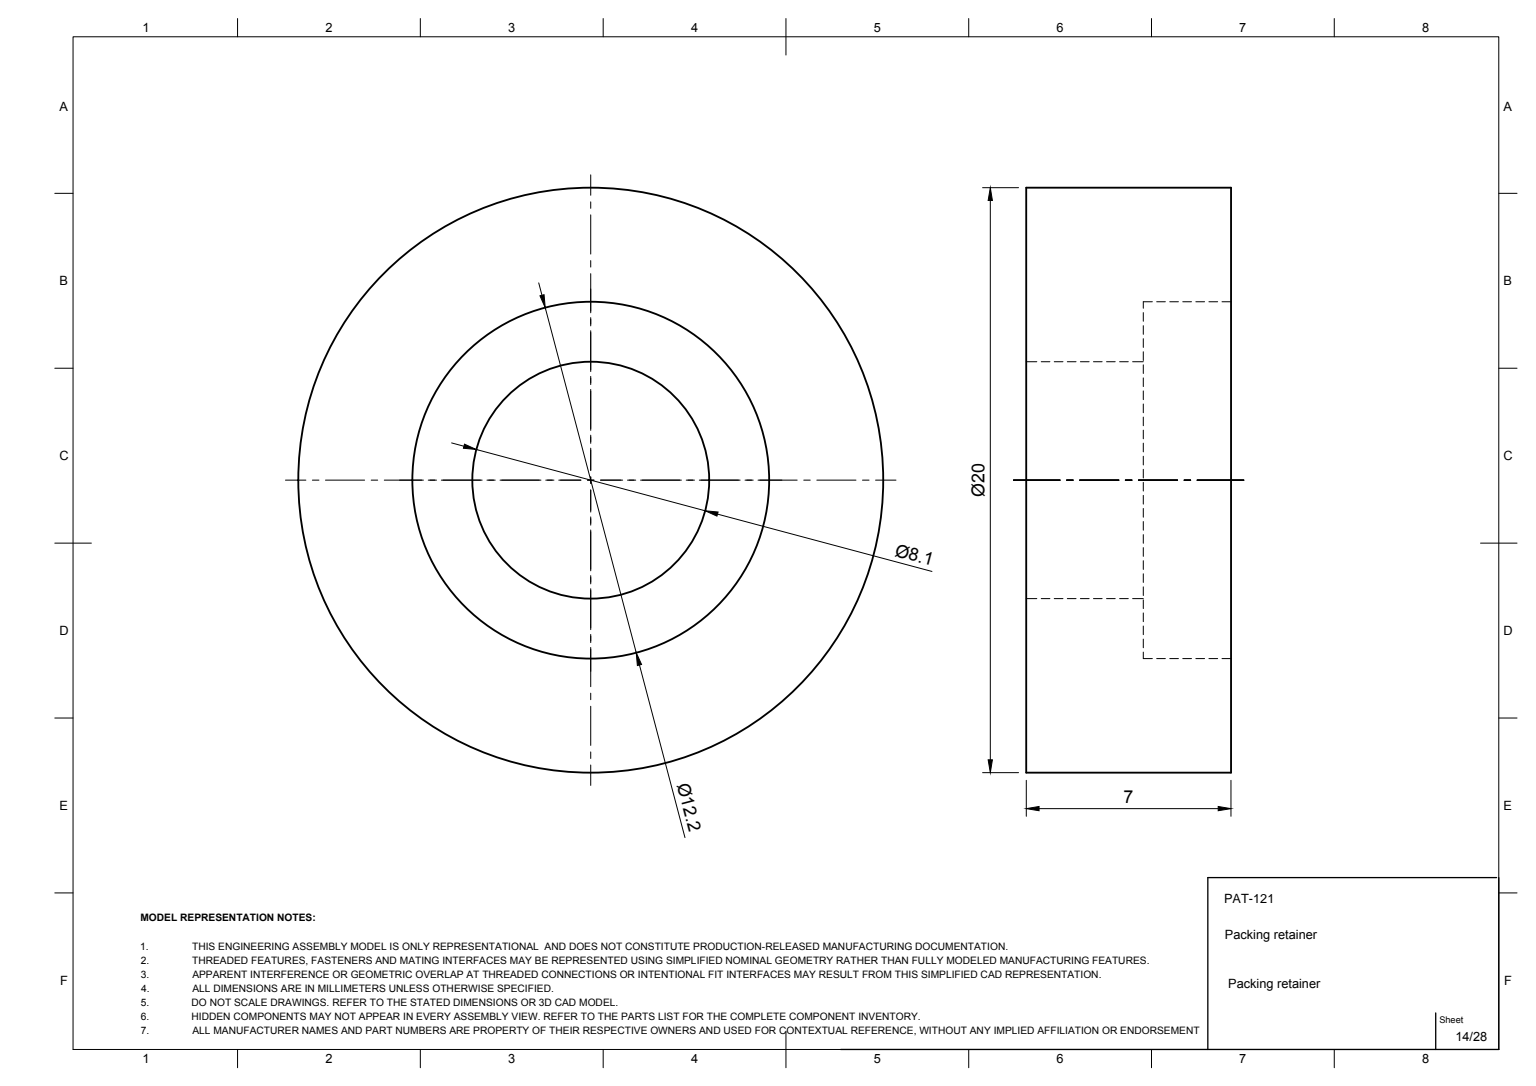
ISO-10303-21;
HEADER;
/* Generated by software containing ST-Developer
 * from STEP Tools, Inc. (www.steptools.com) 
 */

FILE_DESCRIPTION(
/* description */ ('Wall-mounted air drop station'),
/* implementation_level */ '2;1');

FILE_NAME(
/* name */ 'Packing retainer.step',
/* time_stamp */ '2026-10-28T22:16:19-07:00',
/* author */ (''),
/* organization */ (''),
/* preprocessor_version */ 'ST-DEVELOPER v20.2',
/* originating_system */ 'Autodesk Translation Framework v15.17.0.0',
/* authorisation */ '');

FILE_SCHEMA (('AUTOMOTIVE_DESIGN { 1 0 10303 214 3 1 1 }'));
ENDSEC;

DATA;
#10=MECHANICAL_DESIGN_GEOMETRIC_PRESENTATION_REPRESENTATION('',(#354),#10517);
#296=SHAPE_REPRESENTATION_RELATIONSHIP('SRR','None',#10653,#325);
#325=ADVANCED_BREP_SHAPE_REPRESENTATION('',(#383),#10497);
#354=STYLED_ITEM('',(#10860),#383);
#383=MANIFOLD_SOLID_BREP('Body1',#5893);
#474=FACE_BOUND('',#1335,.T.);
#475=FACE_BOUND('',#1339,.T.);
#476=FACE_BOUND('',#1341,.T.);
#616=PLANE('',#6515);
#617=PLANE('',#6522);
#618=PLANE('',#6523);
#903=FACE_OUTER_BOUND('',#1333,.T.);
#904=FACE_OUTER_BOUND('',#1334,.T.);
#905=FACE_OUTER_BOUND('',#1336,.T.);
#906=FACE_OUTER_BOUND('',#1337,.T.);
#907=FACE_OUTER_BOUND('',#1338,.T.);
#908=FACE_OUTER_BOUND('',#1340,.T.);
#1333=EDGE_LOOP('',(#4613,#4614,#4615,#4616));
#1334=EDGE_LOOP('',(#4617));
#1335=EDGE_LOOP('',(#4618));
#1336=EDGE_LOOP('',(#4619,#4620,#4621,#4622));
#1337=EDGE_LOOP('',(#4623,#4624,#4625,#4626));
#1338=EDGE_LOOP('',(#4627));
#1339=EDGE_LOOP('',(#4628));
#1340=EDGE_LOOP('',(#4629));
#1341=EDGE_LOOP('',(#4630));
#1796=LINE('',#9464,#2260);
#1797=LINE('',#9472,#2261);
#1798=LINE('',#9477,#2262);
#2260=VECTOR('',#7686,0.61);
#2261=VECTOR('',#7697,0.405);
#2262=VECTOR('',#7702,1.);
#2636=CIRCLE('',#6513,0.61);
#2637=CIRCLE('',#6514,0.61);
#2638=CIRCLE('',#6516,0.405);
#2639=CIRCLE('',#6518,0.405);
#2640=CIRCLE('',#6520,1.);
#2641=CIRCLE('',#6521,1.);
#2978=VERTEX_POINT('',#9461);
#2979=VERTEX_POINT('',#9463);
#2980=VERTEX_POINT('',#9467);
#2981=VERTEX_POINT('',#9470);
#2982=VERTEX_POINT('',#9474);
#2983=VERTEX_POINT('',#9476);
#3564=EDGE_CURVE('',#2978,#2978,#2636,.T.);
#3565=EDGE_CURVE('',#2978,#2979,#1796,.T.);
#3566=EDGE_CURVE('',#2979,#2979,#2637,.T.);
#3567=EDGE_CURVE('',#2980,#2980,#2638,.T.);
#3568=EDGE_CURVE('',#2981,#2981,#2639,.T.);
#3569=EDGE_CURVE('',#2981,#2980,#1797,.T.);
#3570=EDGE_CURVE('',#2982,#2982,#2640,.T.);
#3571=EDGE_CURVE('',#2982,#2983,#1798,.T.);
#3572=EDGE_CURVE('',#2983,#2983,#2641,.T.);
#4613=ORIENTED_EDGE('',*,*,#3564,.F.);
#4614=ORIENTED_EDGE('',*,*,#3565,.T.);
#4615=ORIENTED_EDGE('',*,*,#3566,.T.);
#4616=ORIENTED_EDGE('',*,*,#3565,.F.);
#4617=ORIENTED_EDGE('',*,*,#3566,.F.);
#4618=ORIENTED_EDGE('',*,*,#3567,.F.);
#4619=ORIENTED_EDGE('',*,*,#3568,.F.);
#4620=ORIENTED_EDGE('',*,*,#3569,.T.);
#4621=ORIENTED_EDGE('',*,*,#3567,.T.);
#4622=ORIENTED_EDGE('',*,*,#3569,.F.);
#4623=ORIENTED_EDGE('',*,*,#3570,.F.);
#4624=ORIENTED_EDGE('',*,*,#3571,.T.);
#4625=ORIENTED_EDGE('',*,*,#3572,.T.);
#4626=ORIENTED_EDGE('',*,*,#3571,.F.);
#4627=ORIENTED_EDGE('',*,*,#3570,.T.);
#4628=ORIENTED_EDGE('',*,*,#3568,.T.);
#4629=ORIENTED_EDGE('',*,*,#3572,.F.);
#4630=ORIENTED_EDGE('',*,*,#3564,.T.);
#5483=CYLINDRICAL_SURFACE('',#6512,0.61);
#5484=CYLINDRICAL_SURFACE('',#6517,0.405);
#5485=CYLINDRICAL_SURFACE('',#6519,1.);
#5676=ADVANCED_FACE('',(#903),#5483,.F.);
#5677=ADVANCED_FACE('',(#904,#474),#616,.F.);
#5678=ADVANCED_FACE('',(#905),#5484,.F.);
#5679=ADVANCED_FACE('',(#906),#5485,.T.);
#5680=ADVANCED_FACE('',(#907,#475),#617,.T.);
#5681=ADVANCED_FACE('',(#908,#476),#618,.F.);
#5893=CLOSED_SHELL('',(#5676,#5677,#5678,#5679,#5680,#5681));
#6511=AXIS2_PLACEMENT_3D('',#9459,#7680,#7681);
#6512=AXIS2_PLACEMENT_3D('',#9460,#7682,#7683);
#6513=AXIS2_PLACEMENT_3D('',#9462,#7684,#7685);
#6514=AXIS2_PLACEMENT_3D('',#9465,#7687,#7688);
#6515=AXIS2_PLACEMENT_3D('',#9466,#7689,#7690);
#6516=AXIS2_PLACEMENT_3D('',#9468,#7691,#7692);
#6517=AXIS2_PLACEMENT_3D('',#9469,#7693,#7694);
#6518=AXIS2_PLACEMENT_3D('',#9471,#7695,#7696);
#6519=AXIS2_PLACEMENT_3D('',#9473,#7698,#7699);
#6520=AXIS2_PLACEMENT_3D('',#9475,#7700,#7701);
#6521=AXIS2_PLACEMENT_3D('',#9478,#7703,#7704);
#6522=AXIS2_PLACEMENT_3D('',#9479,#7705,#7706);
#6523=AXIS2_PLACEMENT_3D('',#9480,#7707,#7708);
#7680=DIRECTION('axis',(0.,0.,1.));
#7681=DIRECTION('refdir',(1.,0.,0.));
#7682=DIRECTION('center_axis',(0.,0.,1.));
#7683=DIRECTION('ref_axis',(1.,0.,0.));
#7684=DIRECTION('center_axis',(0.,0.,1.));
#7685=DIRECTION('ref_axis',(1.,0.,0.));
#7686=DIRECTION('',(0.,0.,1.));
#7687=DIRECTION('center_axis',(0.,0.,1.));
#7688=DIRECTION('ref_axis',(1.,0.,0.));
#7689=DIRECTION('center_axis',(0.,0.,1.));
#7690=DIRECTION('ref_axis',(1.,0.,0.));
#7691=DIRECTION('center_axis',(0.,0.,-1.));
#7692=DIRECTION('ref_axis',(1.,0.,0.));
#7693=DIRECTION('center_axis',(0.,0.,1.));
#7694=DIRECTION('ref_axis',(1.,0.,0.));
#7695=DIRECTION('center_axis',(0.,0.,-1.));
#7696=DIRECTION('ref_axis',(1.,0.,0.));
#7697=DIRECTION('',(0.,0.,-1.));
#7698=DIRECTION('center_axis',(0.,0.,1.));
#7699=DIRECTION('ref_axis',(1.,0.,0.));
#7700=DIRECTION('center_axis',(0.,0.,1.));
#7701=DIRECTION('ref_axis',(1.,0.,0.));
#7702=DIRECTION('',(0.,0.,-1.));
#7703=DIRECTION('center_axis',(0.,0.,1.));
#7704=DIRECTION('ref_axis',(1.,0.,0.));
#7705=DIRECTION('center_axis',(0.,0.,1.));
#7706=DIRECTION('ref_axis',(1.,0.,0.));
#7707=DIRECTION('center_axis',(0.,0.,1.));
#7708=DIRECTION('ref_axis',(1.,0.,0.));
#9459=CARTESIAN_POINT('',(0.,0.,0.));
#9460=CARTESIAN_POINT('Origin',(0.,0.,7.9));
#9461=CARTESIAN_POINT('',(-0.61,-7.47034547479885E-17,8.));
#9462=CARTESIAN_POINT('Origin',(0.,0.,8.));
#9463=CARTESIAN_POINT('',(-0.61,-7.47034547479885E-17,8.3));
#9464=CARTESIAN_POINT('',(-0.61,-7.47034547479885E-17,7.9));
#9465=CARTESIAN_POINT('Origin',(0.,0.,8.3));
#9466=CARTESIAN_POINT('Origin',(0.,0.,8.3));
#9467=CARTESIAN_POINT('',(-0.405,4.95981953654678E-17,8.3));
#9468=CARTESIAN_POINT('Origin',(0.,0.,8.3));
#9469=CARTESIAN_POINT('Origin',(0.,0.,8.));
#9470=CARTESIAN_POINT('',(-0.405,-4.95981953654678E-17,8.7));
#9471=CARTESIAN_POINT('Origin',(0.,0.,8.7));
#9472=CARTESIAN_POINT('',(-0.405,-4.95981953654678E-17,8.));
#9473=CARTESIAN_POINT('Origin',(0.,0.,8.));
#9474=CARTESIAN_POINT('',(-1.,-1.22464679914735E-16,8.7));
#9475=CARTESIAN_POINT('Origin',(0.,0.,8.7));
#9476=CARTESIAN_POINT('',(-1.,-1.22464679914735E-16,8.));
#9477=CARTESIAN_POINT('',(-1.,-1.22464679914735E-16,8.));
#9478=CARTESIAN_POINT('Origin',(0.,0.,8.));
#9479=CARTESIAN_POINT('Origin',(0.,0.,8.7));
#9480=CARTESIAN_POINT('Origin',(0.,0.,8.));
#10464=UNCERTAINTY_MEASURE_WITH_UNIT(LENGTH_MEASURE(0.001),#10518,
'DISTANCE_ACCURACY_VALUE',
'Maximum model space distance between geometric entities at asserted c
onnectivities');
#10484=UNCERTAINTY_MEASURE_WITH_UNIT(LENGTH_MEASURE(0.001),#10518,
'DISTANCE_ACCURACY_VALUE',
'Maximum model space distance between geometric entities at asserted c
onnectivities');
#10497=(
GEOMETRIC_REPRESENTATION_CONTEXT(3)
GLOBAL_UNCERTAINTY_ASSIGNED_CONTEXT((#10464))
GLOBAL_UNIT_ASSIGNED_CONTEXT((#10518,#10520,#10521))
REPRESENTATION_CONTEXT('','3D')
);
#10517=(
GEOMETRIC_REPRESENTATION_CONTEXT(3)
GLOBAL_UNCERTAINTY_ASSIGNED_CONTEXT((#10484))
GLOBAL_UNIT_ASSIGNED_CONTEXT((#10518,#10520,#10521))
REPRESENTATION_CONTEXT('','3D')
);
#10518=(
LENGTH_UNIT()
NAMED_UNIT(*)
SI_UNIT(.CENTI.,.METRE.)
);
#10520=(
NAMED_UNIT(*)
PLANE_ANGLE_UNIT()
SI_UNIT($,.RADIAN.)
);
#10521=(
NAMED_UNIT(*)
SI_UNIT($,.STERADIAN.)
SOLID_ANGLE_UNIT()
);
#10534=SHAPE_DEFINITION_REPRESENTATION(#10566,#10653);
#10566=PRODUCT_DEFINITION_SHAPE('',$,#10686);
#10653=SHAPE_REPRESENTATION('',(#6511),#10497);
#10673=PRODUCT_DEFINITION_CONTEXT('part definition',#10771,'design');
#10686=PRODUCT_DEFINITION('Packing retainer','Packing retainer',#10718,
#10673);
#10718=PRODUCT_DEFINITION_FORMATION('',$,#10785);
#10771=APPLICATION_CONTEXT(
'Core Data for Automotive Mechanical Design Process');
#10772=PRODUCT_CONTEXT('part definition',#10771,'mechanical');
#10785=PRODUCT('Packing retainer','Packing retainer','Packing retainer',
(#10772));
#10854=COLOUR_RGB('Light Blue',0.38,0.62,0.78);
#10855=FILL_AREA_STYLE_COLOUR('',#10854);
#10856=FILL_AREA_STYLE('',(#10855));
#10857=SURFACE_STYLE_FILL_AREA(#10856);
#10858=SURFACE_SIDE_STYLE('',(#10857));
#10859=SURFACE_STYLE_USAGE(.BOTH.,#10858);
#10860=PRESENTATION_STYLE_ASSIGNMENT((#10859));
ENDSEC;
END-ISO-10303-21;
